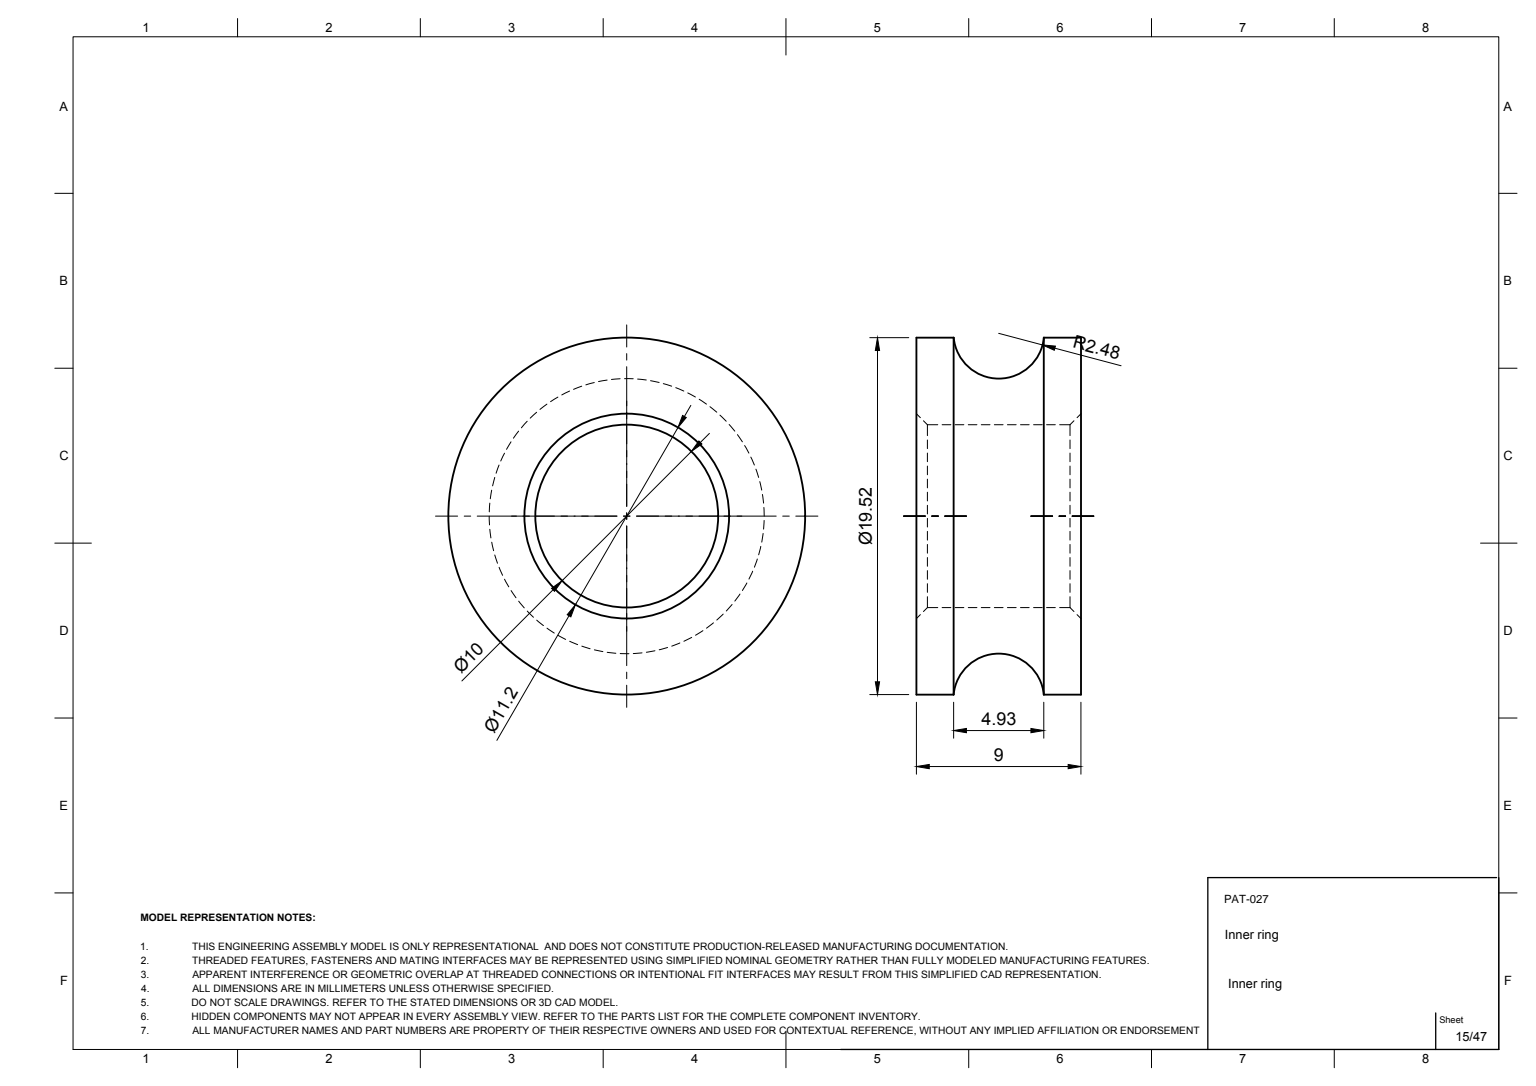
ISO-10303-21;
HEADER;
/* Generated by software containing ST-Developer
 * from STEP Tools, Inc. (www.steptools.com) 
 */

FILE_DESCRIPTION(
/* description */ ('Crank-driven oscillating fan base (mechanism only)'),

/* implementation_level */ '2;1');

FILE_NAME(
/* name */ 'Inner ring.step',
/* time_stamp */ '2026-10-28T03:25:00-07:00',
/* author */ (''),
/* organization */ (''),
/* preprocessor_version */ 'ST-DEVELOPER v20.2',
/* originating_system */ 'Autodesk Translation Framework v15.17.0.0',
/* authorisation */ '');

FILE_SCHEMA (('AUTOMOTIVE_DESIGN { 1 0 10303 214 3 1 1 }'));
ENDSEC;

DATA;
#10=MECHANICAL_DESIGN_GEOMETRIC_PRESENTATION_REPRESENTATION('',(#446),#11916);
#291=TOROIDAL_SURFACE('',#6831,1.,0.247676);
#296=CONICAL_SURFACE('',#6842,0.53,0.785398163397448);
#297=CONICAL_SURFACE('',#6849,0.53,0.785398163397448);
#366=SHAPE_REPRESENTATION_RELATIONSHIP('SRR','None',#12091,#406);
#406=ADVANCED_BREP_SHAPE_REPRESENTATION('',(#493),#11882);
#446=STYLED_ITEM('',(#12375),#493);
#493=MANIFOLD_SOLID_BREP('Body1',#6077);
#607=FACE_BOUND('',#1467,.T.);
#608=FACE_BOUND('',#1470,.T.);
#753=PLANE('',#6844);
#754=PLANE('',#6847);
#1010=FACE_OUTER_BOUND('',#1462,.T.);
#1011=FACE_OUTER_BOUND('',#1463,.T.);
#1012=FACE_OUTER_BOUND('',#1464,.T.);
#1013=FACE_OUTER_BOUND('',#1465,.T.);
#1014=FACE_OUTER_BOUND('',#1466,.T.);
#1015=FACE_OUTER_BOUND('',#1468,.T.);
#1016=FACE_OUTER_BOUND('',#1469,.T.);
#1017=FACE_OUTER_BOUND('',#1471,.T.);
#1462=EDGE_LOOP('',(#4604,#4605,#4606,#4607,#4608,#4609));
#1463=EDGE_LOOP('',(#4610,#4611,#4612,#4613,#4614));
#1464=EDGE_LOOP('',(#4615,#4616,#4617,#4618));
#1465=EDGE_LOOP('',(#4619,#4620,#4621,#4622));
#1466=EDGE_LOOP('',(#4623));
#1467=EDGE_LOOP('',(#4624));
#1468=EDGE_LOOP('',(#4625,#4626,#4627,#4628,#4629));
#1469=EDGE_LOOP('',(#4630));
#1470=EDGE_LOOP('',(#4631));
#1471=EDGE_LOOP('',(#4632,#4633,#4634,#4635));
#1923=LINE('',#10180,#2256);
#1924=LINE('',#10186,#2257);
#1925=LINE('',#10190,#2258);
#1926=LINE('',#10196,#2259);
#1927=LINE('',#10201,#2260);
#2256=VECTOR('',#8094,0.976185);
#2257=VECTOR('',#8101,0.5);
#2258=VECTOR('',#8106,0.53);
#2259=VECTOR('',#8115,0.976185);
#2260=VECTOR('',#8122,0.53);
#2599=CIRCLE('',#6832,0.976185);
#2600=CIRCLE('',#6833,0.976185);
#2601=CIRCLE('',#6834,0.247676);
#2602=CIRCLE('',#6835,0.976185);
#2603=CIRCLE('',#6836,0.976185);
#2604=CIRCLE('',#6838,0.976185);
#2605=CIRCLE('',#6840,0.5);
#2606=CIRCLE('',#6841,0.5);
#2607=CIRCLE('',#6843,0.56);
#2608=CIRCLE('',#6846,0.976185);
#2609=CIRCLE('',#6848,0.56);
#3008=VERTEX_POINT('',#10169);
#3009=VERTEX_POINT('',#10170);
#3010=VERTEX_POINT('',#10173);
#3011=VERTEX_POINT('',#10175);
#3012=VERTEX_POINT('',#10179);
#3013=VERTEX_POINT('',#10183);
#3014=VERTEX_POINT('',#10185);
#3015=VERTEX_POINT('',#10189);
#3016=VERTEX_POINT('',#10194);
#3017=VERTEX_POINT('',#10198);
#3597=EDGE_CURVE('',#3008,#3009,#2599,.T.);
#3598=EDGE_CURVE('',#3009,#3008,#2600,.T.);
#3599=EDGE_CURVE('',#3009,#3010,#2601,.T.);
#3600=EDGE_CURVE('',#3011,#3010,#2602,.T.);
#3601=EDGE_CURVE('',#3010,#3011,#2603,.T.);
#3602=EDGE_CURVE('',#3011,#3012,#1923,.T.);
#3603=EDGE_CURVE('',#3012,#3012,#2604,.T.);
#3604=EDGE_CURVE('',#3013,#3013,#2605,.T.);
#3605=EDGE_CURVE('',#3013,#3014,#1924,.T.);
#3606=EDGE_CURVE('',#3014,#3014,#2606,.T.);
#3607=EDGE_CURVE('',#3014,#3015,#1925,.T.);
#3608=EDGE_CURVE('',#3015,#3015,#2607,.T.);
#3609=EDGE_CURVE('',#3016,#3016,#2608,.T.);
#3610=EDGE_CURVE('',#3016,#3008,#1926,.T.);
#3611=EDGE_CURVE('',#3017,#3017,#2609,.T.);
#3612=EDGE_CURVE('',#3017,#3013,#1927,.T.);
#4604=ORIENTED_EDGE('',*,*,#3597,.F.);
#4605=ORIENTED_EDGE('',*,*,#3598,.F.);
#4606=ORIENTED_EDGE('',*,*,#3599,.T.);
#4607=ORIENTED_EDGE('',*,*,#3600,.F.);
#4608=ORIENTED_EDGE('',*,*,#3601,.F.);
#4609=ORIENTED_EDGE('',*,*,#3599,.F.);
#4610=ORIENTED_EDGE('',*,*,#3600,.T.);
#4611=ORIENTED_EDGE('',*,*,#3601,.T.);
#4612=ORIENTED_EDGE('',*,*,#3602,.T.);
#4613=ORIENTED_EDGE('',*,*,#3603,.T.);
#4614=ORIENTED_EDGE('',*,*,#3602,.F.);
#4615=ORIENTED_EDGE('',*,*,#3604,.T.);
#4616=ORIENTED_EDGE('',*,*,#3605,.T.);
#4617=ORIENTED_EDGE('',*,*,#3606,.F.);
#4618=ORIENTED_EDGE('',*,*,#3605,.F.);
#4619=ORIENTED_EDGE('',*,*,#3606,.T.);
#4620=ORIENTED_EDGE('',*,*,#3607,.T.);
#4621=ORIENTED_EDGE('',*,*,#3608,.F.);
#4622=ORIENTED_EDGE('',*,*,#3607,.F.);
#4623=ORIENTED_EDGE('',*,*,#3603,.F.);
#4624=ORIENTED_EDGE('',*,*,#3608,.T.);
#4625=ORIENTED_EDGE('',*,*,#3609,.F.);
#4626=ORIENTED_EDGE('',*,*,#3610,.T.);
#4627=ORIENTED_EDGE('',*,*,#3597,.T.);
#4628=ORIENTED_EDGE('',*,*,#3598,.T.);
#4629=ORIENTED_EDGE('',*,*,#3610,.F.);
#4630=ORIENTED_EDGE('',*,*,#3609,.T.);
#4631=ORIENTED_EDGE('',*,*,#3611,.F.);
#4632=ORIENTED_EDGE('',*,*,#3611,.T.);
#4633=ORIENTED_EDGE('',*,*,#3612,.T.);
#4634=ORIENTED_EDGE('',*,*,#3604,.F.);
#4635=ORIENTED_EDGE('',*,*,#3612,.F.);
#5606=CYLINDRICAL_SURFACE('',#6837,0.976185);
#5607=CYLINDRICAL_SURFACE('',#6839,0.5);
#5608=CYLINDRICAL_SURFACE('',#6845,0.976185);
#5816=ADVANCED_FACE('',(#1010),#291,.F.);
#5817=ADVANCED_FACE('',(#1011),#5606,.T.);
#5818=ADVANCED_FACE('',(#1012),#5607,.F.);
#5819=ADVANCED_FACE('',(#1013),#296,.F.);
#5820=ADVANCED_FACE('',(#1014,#607),#753,.T.);
#5821=ADVANCED_FACE('',(#1015),#5608,.T.);
#5822=ADVANCED_FACE('',(#1016,#608),#754,.T.);
#5823=ADVANCED_FACE('',(#1017),#297,.F.);
#6077=CLOSED_SHELL('',(#5816,#5817,#5818,#5819,#5820,#5821,#5822,#5823));
#6830=AXIS2_PLACEMENT_3D('',#10167,#8078,#8079);
#6831=AXIS2_PLACEMENT_3D('',#10168,#8080,#8081);
#6832=AXIS2_PLACEMENT_3D('',#10171,#8082,#8083);
#6833=AXIS2_PLACEMENT_3D('',#10172,#8084,#8085);
#6834=AXIS2_PLACEMENT_3D('',#10174,#8086,#8087);
#6835=AXIS2_PLACEMENT_3D('',#10176,#8088,#8089);
#6836=AXIS2_PLACEMENT_3D('',#10177,#8090,#8091);
#6837=AXIS2_PLACEMENT_3D('',#10178,#8092,#8093);
#6838=AXIS2_PLACEMENT_3D('',#10181,#8095,#8096);
#6839=AXIS2_PLACEMENT_3D('',#10182,#8097,#8098);
#6840=AXIS2_PLACEMENT_3D('',#10184,#8099,#8100);
#6841=AXIS2_PLACEMENT_3D('',#10187,#8102,#8103);
#6842=AXIS2_PLACEMENT_3D('',#10188,#8104,#8105);
#6843=AXIS2_PLACEMENT_3D('',#10191,#8107,#8108);
#6844=AXIS2_PLACEMENT_3D('',#10192,#8109,#8110);
#6845=AXIS2_PLACEMENT_3D('',#10193,#8111,#8112);
#6846=AXIS2_PLACEMENT_3D('',#10195,#8113,#8114);
#6847=AXIS2_PLACEMENT_3D('',#10197,#8116,#8117);
#6848=AXIS2_PLACEMENT_3D('',#10199,#8118,#8119);
#6849=AXIS2_PLACEMENT_3D('',#10200,#8120,#8121);
#8078=DIRECTION('axis',(0.,0.,1.));
#8079=DIRECTION('refdir',(1.,0.,0.));
#8080=DIRECTION('center_axis',(0.,-1.,0.));
#8081=DIRECTION('ref_axis',(0.,0.,-1.));
#8082=DIRECTION('center_axis',(0.,-1.,0.));
#8083=DIRECTION('ref_axis',(1.,0.,0.));
#8084=DIRECTION('center_axis',(0.,-1.,0.));
#8085=DIRECTION('ref_axis',(1.,0.,0.));
#8086=DIRECTION('center_axis',(1.,0.,1.22464679914735E-16));
#8087=DIRECTION('ref_axis',(-1.22464679914735E-16,0.,1.));
#8088=DIRECTION('center_axis',(0.,1.,0.));
#8089=DIRECTION('ref_axis',(1.,0.,0.));
#8090=DIRECTION('center_axis',(0.,1.,0.));
#8091=DIRECTION('ref_axis',(1.,0.,0.));
#8092=DIRECTION('center_axis',(0.,-1.,0.));
#8093=DIRECTION('ref_axis',(1.,0.,0.));
#8094=DIRECTION('',(0.,1.,0.));
#8095=DIRECTION('center_axis',(0.,-1.,0.));
#8096=DIRECTION('ref_axis',(1.,0.,0.));
#8097=DIRECTION('center_axis',(0.,-1.,0.));
#8098=DIRECTION('ref_axis',(1.,0.,0.));
#8099=DIRECTION('center_axis',(0.,-1.,0.));
#8100=DIRECTION('ref_axis',(1.,0.,0.));
#8101=DIRECTION('',(0.,1.,0.));
#8102=DIRECTION('center_axis',(0.,-1.,0.));
#8103=DIRECTION('ref_axis',(1.,0.,0.));
#8104=DIRECTION('center_axis',(0.,1.,0.));
#8105=DIRECTION('ref_axis',(1.,0.,0.));
#8106=DIRECTION('',(-0.707106781186547,0.707106781186548,-8.65956056235493E-17));
#8107=DIRECTION('center_axis',(0.,-1.,0.));
#8108=DIRECTION('ref_axis',(1.,0.,0.));
#8109=DIRECTION('center_axis',(0.,1.,0.));
#8110=DIRECTION('ref_axis',(0.,0.,1.));
#8111=DIRECTION('center_axis',(0.,-1.,0.));
#8112=DIRECTION('ref_axis',(1.,0.,0.));
#8113=DIRECTION('center_axis',(0.,-1.,0.));
#8114=DIRECTION('ref_axis',(1.,0.,0.));
#8115=DIRECTION('',(0.,1.,0.));
#8116=DIRECTION('center_axis',(0.,-1.,0.));
#8117=DIRECTION('ref_axis',(0.,0.,-1.));
#8118=DIRECTION('center_axis',(0.,-1.,0.));
#8119=DIRECTION('ref_axis',(1.,0.,0.));
#8120=DIRECTION('center_axis',(0.,-1.,0.));
#8121=DIRECTION('ref_axis',(1.,0.,0.));
#8122=DIRECTION('',(0.707106781186547,0.707106781186548,8.65956056235493E-17));
#10167=CARTESIAN_POINT('',(0.,0.,0.));
#10168=CARTESIAN_POINT('Origin',(0.,0.,0.));
#10169=CARTESIAN_POINT('',(-0.976185,-0.246528389340863,-1.19548183562566E-16));
#10170=CARTESIAN_POINT('',(-1.19548183562566E-16,-0.246528389340863,0.976185));
#10171=CARTESIAN_POINT('Origin',(0.,-0.246528389340863,0.));
#10172=CARTESIAN_POINT('Origin',(0.,-0.246528389340863,0.));
#10173=CARTESIAN_POINT('',(-1.19548183562566E-16,0.246528389340863,0.976185));
#10174=CARTESIAN_POINT('Origin',(-1.22464679914735E-16,0.,1.));
#10175=CARTESIAN_POINT('',(-0.976185,0.246528389340863,1.19548183562566E-16));
#10176=CARTESIAN_POINT('Origin',(0.,0.246528389340863,0.));
#10177=CARTESIAN_POINT('Origin',(0.,0.246528389340863,0.));
#10178=CARTESIAN_POINT('Origin',(0.,0.,0.));
#10179=CARTESIAN_POINT('',(-0.976185,0.45,-1.19548183562566E-16));
#10180=CARTESIAN_POINT('',(-0.976185,0.,-1.19548183562566E-16));
#10181=CARTESIAN_POINT('Origin',(0.,0.45,0.));
#10182=CARTESIAN_POINT('Origin',(0.,0.,0.));
#10183=CARTESIAN_POINT('',(-0.5,-0.39,-6.12323399573677E-17));
#10184=CARTESIAN_POINT('Origin',(0.,-0.39,0.));
#10185=CARTESIAN_POINT('',(-0.5,0.39,-6.12323399573677E-17));
#10186=CARTESIAN_POINT('',(-0.5,0.,-6.12323399573677E-17));
#10187=CARTESIAN_POINT('Origin',(0.,0.39,0.));
#10188=CARTESIAN_POINT('Origin',(0.,0.42,0.));
#10189=CARTESIAN_POINT('',(-0.56,0.45,-6.85802207522518E-17));
#10190=CARTESIAN_POINT('',(-0.53,0.42,-6.49062803548097E-17));
#10191=CARTESIAN_POINT('Origin',(0.,0.45,0.));
#10192=CARTESIAN_POINT('Origin',(0.976185,0.45,0.));
#10193=CARTESIAN_POINT('Origin',(0.,0.,0.));
#10194=CARTESIAN_POINT('',(-0.976185,-0.45,-1.19548183562566E-16));
#10195=CARTESIAN_POINT('Origin',(0.,-0.45,0.));
#10196=CARTESIAN_POINT('',(-0.976185,0.,-1.19548183562566E-16));
#10197=CARTESIAN_POINT('Origin',(0.56,-0.45,0.));
#10198=CARTESIAN_POINT('',(-0.56,-0.45,-6.85802207522518E-17));
#10199=CARTESIAN_POINT('Origin',(0.,-0.45,0.));
#10200=CARTESIAN_POINT('Origin',(0.,-0.42,0.));
#10201=CARTESIAN_POINT('',(-0.53,-0.42,-6.49062803548097E-17));
#11835=UNCERTAINTY_MEASURE_WITH_UNIT(LENGTH_MEASURE(0.001),#11917,
'DISTANCE_ACCURACY_VALUE',
'Maximum model space distance between geometric entities at asserted c
onnectivities');
#11869=UNCERTAINTY_MEASURE_WITH_UNIT(LENGTH_MEASURE(0.001),#11917,
'DISTANCE_ACCURACY_VALUE',
'Maximum model space distance between geometric entities at asserted c
onnectivities');
#11882=(
GEOMETRIC_REPRESENTATION_CONTEXT(3)
GLOBAL_UNCERTAINTY_ASSIGNED_CONTEXT((#11835))
GLOBAL_UNIT_ASSIGNED_CONTEXT((#11917,#11919,#11920))
REPRESENTATION_CONTEXT('','3D')
);
#11916=(
GEOMETRIC_REPRESENTATION_CONTEXT(3)
GLOBAL_UNCERTAINTY_ASSIGNED_CONTEXT((#11869))
GLOBAL_UNIT_ASSIGNED_CONTEXT((#11917,#11919,#11920))
REPRESENTATION_CONTEXT('','3D')
);
#11917=(
LENGTH_UNIT()
NAMED_UNIT(*)
SI_UNIT(.CENTI.,.METRE.)
);
#11919=(
NAMED_UNIT(*)
PLANE_ANGLE_UNIT()
SI_UNIT($,.RADIAN.)
);
#11920=(
NAMED_UNIT(*)
SI_UNIT($,.STERADIAN.)
SOLID_ANGLE_UNIT()
);
#11933=SHAPE_DEFINITION_REPRESENTATION(#11979,#12091);
#11979=PRODUCT_DEFINITION_SHAPE('',$,#12138);
#12091=SHAPE_REPRESENTATION('',(#6830),#11882);
#12125=PRODUCT_DEFINITION_CONTEXT('part definition',#12265,'design');
#12138=PRODUCT_DEFINITION('Inner ring','Inner ring',#12184,#12125);
#12184=PRODUCT_DEFINITION_FORMATION('',$,#12279);
#12265=APPLICATION_CONTEXT(
'Core Data for Automotive Mechanical Design Process');
#12266=PRODUCT_CONTEXT('part definition',#12265,'mechanical');
#12279=PRODUCT('Inner ring','Inner ring','Inner ring',(#12266));
#12369=COLOUR_RGB('Grey',0.48,0.52,0.57);
#12370=FILL_AREA_STYLE_COLOUR('',#12369);
#12371=FILL_AREA_STYLE('',(#12370));
#12372=SURFACE_STYLE_FILL_AREA(#12371);
#12373=SURFACE_SIDE_STYLE('',(#12372));
#12374=SURFACE_STYLE_USAGE(.BOTH.,#12373);
#12375=PRESENTATION_STYLE_ASSIGNMENT((#12374));
ENDSEC;
END-ISO-10303-21;
